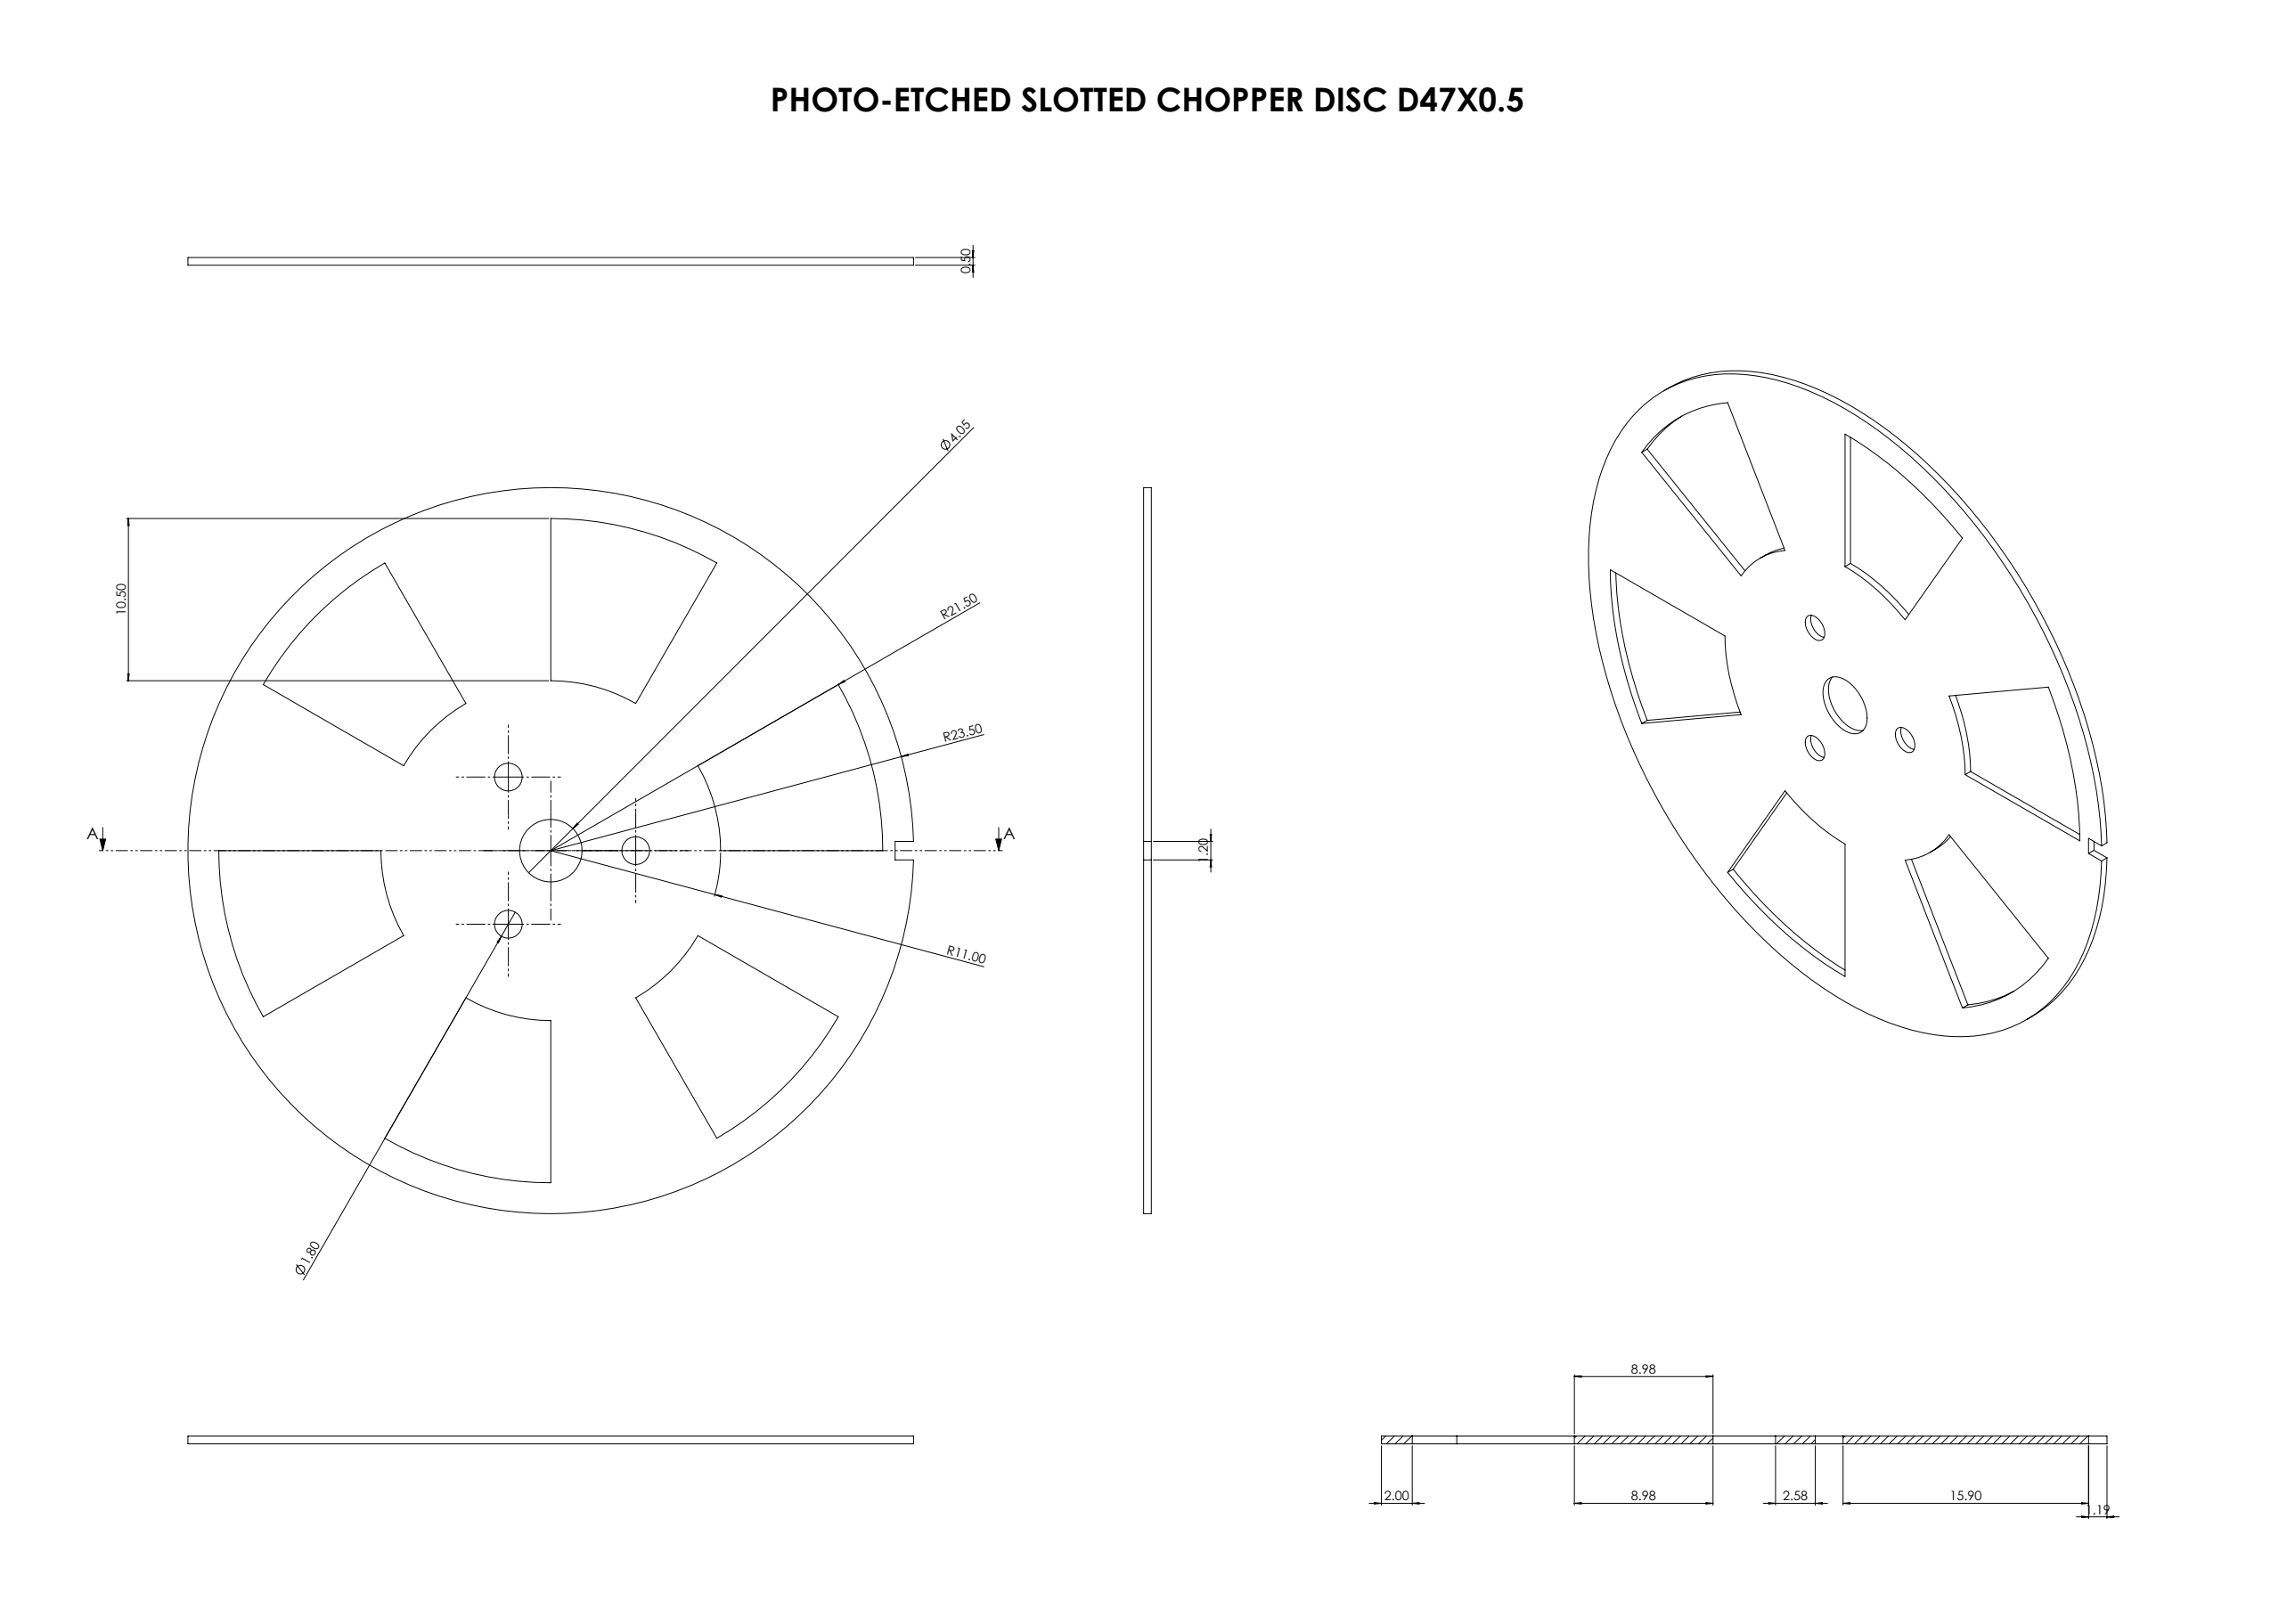
ISO-10303-21;
HEADER;
/* Generated by software containing ST-Developer
 * from STEP Tools, Inc. (www.steptools.com) 
 */

FILE_DESCRIPTION(
/* description */ (''),
/* implementation_level */ '2;1');

FILE_NAME(
/* name */ '10_Photo-Etched_Slotted_Chopper_Disc_D47x0.5.step',
/* time_stamp */ '2026-10-19T23:00:43-07:00',
/* author */ (''),
/* organization */ (''),
/* preprocessor_version */ 'ST-DEVELOPER v20.2',
/* originating_system */ 'Autodesk Translation Framework v15.15.0.0',
/* authorisation */ '');

FILE_SCHEMA (('AUTOMOTIVE_DESIGN { 1 0 10303 214 3 1 1 }'));
ENDSEC;

DATA;
#10=MECHANICAL_DESIGN_GEOMETRIC_PRESENTATION_REPRESENTATION('',(#1005),#55002);
#965=SHAPE_REPRESENTATION_RELATIONSHIP('SRR','None',#55113,#985);
#985=ADVANCED_BREP_SHAPE_REPRESENTATION('',(#1025),#54991);
#1005=STYLED_ITEM('',(#55379),#1025);
#1025=MANIFOLD_SOLID_BREP('Chopper Disc',#24538);
#1212=FACE_BOUND('',#4510,.T.);
#1213=FACE_BOUND('',#4511,.T.);
#1214=FACE_BOUND('',#4512,.T.);
#1215=FACE_BOUND('',#4513,.T.);
#1216=FACE_BOUND('',#4514,.T.);
#1217=FACE_BOUND('',#4515,.T.);
#1218=FACE_BOUND('',#4516,.T.);
#1219=FACE_BOUND('',#4517,.T.);
#1220=FACE_BOUND('',#4518,.T.);
#1221=FACE_BOUND('',#4519,.T.);
#1222=FACE_BOUND('',#4550,.T.);
#1223=FACE_BOUND('',#4551,.T.);
#1224=FACE_BOUND('',#4552,.T.);
#1225=FACE_BOUND('',#4553,.T.);
#1226=FACE_BOUND('',#4554,.T.);
#1227=FACE_BOUND('',#4555,.T.);
#1228=FACE_BOUND('',#4556,.T.);
#1229=FACE_BOUND('',#4557,.T.);
#1230=FACE_BOUND('',#4558,.T.);
#1231=FACE_BOUND('',#4559,.T.);
#1441=PLANE('',#25954);
#1442=PLANE('',#25955);
#1443=PLANE('',#25956);
#1444=PLANE('',#25957);
#1445=PLANE('',#25983);
#1446=PLANE('',#25986);
#1447=PLANE('',#25989);
#1448=PLANE('',#25992);
#1449=PLANE('',#25995);
#1450=PLANE('',#25998);
#1451=PLANE('',#26001);
#1452=PLANE('',#26004);
#1453=PLANE('',#26007);
#1454=PLANE('',#26010);
#1455=PLANE('',#26013);
#1456=PLANE('',#26016);
#1457=PLANE('',#26021);
#2161=CYLINDRICAL_SURFACE('',#25975,2.35);
#2162=CYLINDRICAL_SURFACE('',#25977,0.09);
#2163=CYLINDRICAL_SURFACE('',#25979,0.09);
#2164=CYLINDRICAL_SURFACE('',#25981,0.0900000000000001);
#2165=CYLINDRICAL_SURFACE('',#25984,1.1);
#2166=CYLINDRICAL_SURFACE('',#25987,2.15);
#2167=CYLINDRICAL_SURFACE('',#25990,1.1);
#2168=CYLINDRICAL_SURFACE('',#25993,2.15);
#2169=CYLINDRICAL_SURFACE('',#25996,1.1);
#2170=CYLINDRICAL_SURFACE('',#25999,2.15);
#2171=CYLINDRICAL_SURFACE('',#26002,1.1);
#2172=CYLINDRICAL_SURFACE('',#26005,2.15);
#2173=CYLINDRICAL_SURFACE('',#26008,1.1);
#2174=CYLINDRICAL_SURFACE('',#26011,2.15);
#2175=CYLINDRICAL_SURFACE('',#26014,1.1);
#2176=CYLINDRICAL_SURFACE('',#26017,2.15);
#2177=CYLINDRICAL_SURFACE('',#26019,0.2025);
#2966=FACE_OUTER_BOUND('',#4506,.T.);
#2967=FACE_OUTER_BOUND('',#4507,.T.);
#2968=FACE_OUTER_BOUND('',#4508,.T.);
#2969=FACE_OUTER_BOUND('',#4509,.T.);
#2970=FACE_OUTER_BOUND('',#4520,.T.);
#2971=FACE_OUTER_BOUND('',#4521,.T.);
#2972=FACE_OUTER_BOUND('',#4522,.T.);
#2973=FACE_OUTER_BOUND('',#4523,.T.);
#2974=FACE_OUTER_BOUND('',#4524,.T.);
#2975=FACE_OUTER_BOUND('',#4525,.T.);
#2976=FACE_OUTER_BOUND('',#4526,.T.);
#2977=FACE_OUTER_BOUND('',#4527,.T.);
#2978=FACE_OUTER_BOUND('',#4528,.T.);
#2979=FACE_OUTER_BOUND('',#4529,.T.);
#2980=FACE_OUTER_BOUND('',#4530,.T.);
#2981=FACE_OUTER_BOUND('',#4531,.T.);
#2982=FACE_OUTER_BOUND('',#4532,.T.);
#2983=FACE_OUTER_BOUND('',#4533,.T.);
#2984=FACE_OUTER_BOUND('',#4534,.T.);
#2985=FACE_OUTER_BOUND('',#4535,.T.);
#2986=FACE_OUTER_BOUND('',#4536,.T.);
#2987=FACE_OUTER_BOUND('',#4537,.T.);
#2988=FACE_OUTER_BOUND('',#4538,.T.);
#2989=FACE_OUTER_BOUND('',#4539,.T.);
#2990=FACE_OUTER_BOUND('',#4540,.T.);
#2991=FACE_OUTER_BOUND('',#4541,.T.);
#2992=FACE_OUTER_BOUND('',#4542,.T.);
#2993=FACE_OUTER_BOUND('',#4543,.T.);
#2994=FACE_OUTER_BOUND('',#4544,.T.);
#2995=FACE_OUTER_BOUND('',#4545,.T.);
#2996=FACE_OUTER_BOUND('',#4546,.T.);
#2997=FACE_OUTER_BOUND('',#4547,.T.);
#2998=FACE_OUTER_BOUND('',#4548,.T.);
#2999=FACE_OUTER_BOUND('',#4549,.T.);
#4506=EDGE_LOOP('',(#18412,#18413,#18414,#18415));
#4507=EDGE_LOOP('',(#18416,#18417,#18418,#18419));
#4508=EDGE_LOOP('',(#18420,#18421,#18422,#18423));
#4509=EDGE_LOOP('',(#18424,#18425,#18426,#18427));
#4510=EDGE_LOOP('',(#18428));
#4511=EDGE_LOOP('',(#18429));
#4512=EDGE_LOOP('',(#18430));
#4513=EDGE_LOOP('',(#18431,#18432,#18433,#18434));
#4514=EDGE_LOOP('',(#18435,#18436,#18437,#18438));
#4515=EDGE_LOOP('',(#18439,#18440,#18441,#18442));
#4516=EDGE_LOOP('',(#18443,#18444,#18445,#18446));
#4517=EDGE_LOOP('',(#18447,#18448,#18449,#18450));
#4518=EDGE_LOOP('',(#18451,#18452,#18453,#18454));
#4519=EDGE_LOOP('',(#18455));
#4520=EDGE_LOOP('',(#18456,#18457,#18458,#18459));
#4521=EDGE_LOOP('',(#18460,#18461,#18462,#18463));
#4522=EDGE_LOOP('',(#18464,#18465,#18466,#18467));
#4523=EDGE_LOOP('',(#18468,#18469,#18470,#18471));
#4524=EDGE_LOOP('',(#18472,#18473,#18474,#18475));
#4525=EDGE_LOOP('',(#18476,#18477,#18478,#18479));
#4526=EDGE_LOOP('',(#18480,#18481,#18482,#18483));
#4527=EDGE_LOOP('',(#18484,#18485,#18486,#18487));
#4528=EDGE_LOOP('',(#18488,#18489,#18490,#18491));
#4529=EDGE_LOOP('',(#18492,#18493,#18494,#18495));
#4530=EDGE_LOOP('',(#18496,#18497,#18498,#18499));
#4531=EDGE_LOOP('',(#18500,#18501,#18502,#18503));
#4532=EDGE_LOOP('',(#18504,#18505,#18506,#18507));
#4533=EDGE_LOOP('',(#18508,#18509,#18510,#18511));
#4534=EDGE_LOOP('',(#18512,#18513,#18514,#18515));
#4535=EDGE_LOOP('',(#18516,#18517,#18518,#18519));
#4536=EDGE_LOOP('',(#18520,#18521,#18522,#18523));
#4537=EDGE_LOOP('',(#18524,#18525,#18526,#18527));
#4538=EDGE_LOOP('',(#18528,#18529,#18530,#18531));
#4539=EDGE_LOOP('',(#18532,#18533,#18534,#18535));
#4540=EDGE_LOOP('',(#18536,#18537,#18538,#18539));
#4541=EDGE_LOOP('',(#18540,#18541,#18542,#18543));
#4542=EDGE_LOOP('',(#18544,#18545,#18546,#18547));
#4543=EDGE_LOOP('',(#18548,#18549,#18550,#18551));
#4544=EDGE_LOOP('',(#18552,#18553,#18554,#18555));
#4545=EDGE_LOOP('',(#18556,#18557,#18558,#18559));
#4546=EDGE_LOOP('',(#18560,#18561,#18562,#18563));
#4547=EDGE_LOOP('',(#18564,#18565,#18566,#18567));
#4548=EDGE_LOOP('',(#18568,#18569,#18570,#18571));
#4549=EDGE_LOOP('',(#18572,#18573,#18574,#18575));
#4550=EDGE_LOOP('',(#18576));
#4551=EDGE_LOOP('',(#18577));
#4552=EDGE_LOOP('',(#18578));
#4553=EDGE_LOOP('',(#18579,#18580,#18581,#18582));
#4554=EDGE_LOOP('',(#18583,#18584,#18585,#18586));
#4555=EDGE_LOOP('',(#18587,#18588,#18589,#18590));
#4556=EDGE_LOOP('',(#18591,#18592,#18593,#18594));
#4557=EDGE_LOOP('',(#18595,#18596,#18597,#18598));
#4558=EDGE_LOOP('',(#18599,#18600,#18601,#18602));
#4559=EDGE_LOOP('',(#18603));
#6000=LINE('',#37069,#7821);
#6001=LINE('',#37071,#7822);
#6002=LINE('',#37073,#7823);
#6003=LINE('',#37074,#7824);
#6004=LINE('',#37078,#7825);
#6005=LINE('',#37080,#7826);
#6006=LINE('',#37082,#7827);
#6007=LINE('',#37083,#7828);
#6008=LINE('',#37085,#7829);
#6009=LINE('',#37086,#7830);
#6010=LINE('',#37097,#7831);
#6011=LINE('',#37101,#7832);
#6012=LINE('',#37105,#7833);
#6013=LINE('',#37109,#7834);
#6014=LINE('',#37113,#7835);
#6015=LINE('',#37117,#7836);
#6016=LINE('',#37121,#7837);
#6017=LINE('',#37125,#7838);
#6018=LINE('',#37129,#7839);
#6019=LINE('',#37133,#7840);
#6020=LINE('',#37137,#7841);
#6021=LINE('',#37141,#7842);
#6022=LINE('',#37150,#7843);
#6023=LINE('',#37154,#7844);
#6024=LINE('',#37158,#7845);
#6025=LINE('',#37161,#7846);
#6026=LINE('',#37163,#7847);
#6027=LINE('',#37164,#7848);
#6028=LINE('',#37167,#7849);
#6029=LINE('',#37171,#7850);
#6030=LINE('',#37172,#7851);
#6031=LINE('',#37177,#7852);
#6032=LINE('',#37179,#7853);
#6033=LINE('',#37180,#7854);
#6034=LINE('',#37183,#7855);
#6035=LINE('',#37187,#7856);
#6036=LINE('',#37188,#7857);
#6037=LINE('',#37193,#7858);
#6038=LINE('',#37195,#7859);
#6039=LINE('',#37196,#7860);
#6040=LINE('',#37199,#7861);
#6041=LINE('',#37203,#7862);
#6042=LINE('',#37204,#7863);
#6043=LINE('',#37209,#7864);
#6044=LINE('',#37211,#7865);
#6045=LINE('',#37212,#7866);
#6046=LINE('',#37215,#7867);
#6047=LINE('',#37219,#7868);
#6048=LINE('',#37220,#7869);
#6049=LINE('',#37225,#7870);
#6050=LINE('',#37227,#7871);
#6051=LINE('',#37228,#7872);
#6052=LINE('',#37231,#7873);
#6053=LINE('',#37235,#7874);
#6054=LINE('',#37236,#7875);
#6055=LINE('',#37241,#7876);
#6056=LINE('',#37243,#7877);
#6057=LINE('',#37244,#7878);
#6058=LINE('',#37247,#7879);
#6059=LINE('',#37251,#7880);
#6060=LINE('',#37252,#7881);
#6061=LINE('',#37258,#7882);
#7821=VECTOR('',#30186,1.);
#7822=VECTOR('',#30187,1.);
#7823=VECTOR('',#30188,1.);
#7824=VECTOR('',#30189,1.);
#7825=VECTOR('',#30192,1.);
#7826=VECTOR('',#30193,1.);
#7827=VECTOR('',#30194,1.);
#7828=VECTOR('',#30195,1.);
#7829=VECTOR('',#30198,1.);
#7830=VECTOR('',#30199,1.);
#7831=VECTOR('',#30210,1.);
#7832=VECTOR('',#30213,1.);
#7833=VECTOR('',#30216,1.);
#7834=VECTOR('',#30219,1.);
#7835=VECTOR('',#30222,1.);
#7836=VECTOR('',#30225,1.);
#7837=VECTOR('',#30228,1.);
#7838=VECTOR('',#30231,1.);
#7839=VECTOR('',#30234,1.);
#7840=VECTOR('',#30237,1.);
#7841=VECTOR('',#30240,1.);
#7842=VECTOR('',#30243,1.);
#7843=VECTOR('',#30256,0.09);
#7844=VECTOR('',#30261,0.09);
#7845=VECTOR('',#30266,0.0900000000000001);
#7846=VECTOR('',#30269,1.);
#7847=VECTOR('',#30270,1.);
#7848=VECTOR('',#30271,1.);
#7849=VECTOR('',#30274,1.);
#7850=VECTOR('',#30279,1.);
#7851=VECTOR('',#30280,1.);
#7852=VECTOR('',#30287,1.);
#7853=VECTOR('',#30288,1.);
#7854=VECTOR('',#30289,1.);
#7855=VECTOR('',#30292,1.);
#7856=VECTOR('',#30297,1.);
#7857=VECTOR('',#30298,1.);
#7858=VECTOR('',#30305,1.);
#7859=VECTOR('',#30306,1.);
#7860=VECTOR('',#30307,1.);
#7861=VECTOR('',#30310,1.);
#7862=VECTOR('',#30315,1.);
#7863=VECTOR('',#30316,1.);
#7864=VECTOR('',#30323,1.);
#7865=VECTOR('',#30324,1.);
#7866=VECTOR('',#30325,1.);
#7867=VECTOR('',#30328,1.);
#7868=VECTOR('',#30333,1.);
#7869=VECTOR('',#30334,1.);
#7870=VECTOR('',#30341,1.);
#7871=VECTOR('',#30342,1.);
#7872=VECTOR('',#30343,1.);
#7873=VECTOR('',#30346,1.);
#7874=VECTOR('',#30351,1.);
#7875=VECTOR('',#30352,1.);
#7876=VECTOR('',#30359,1.);
#7877=VECTOR('',#30360,1.);
#7878=VECTOR('',#30361,1.);
#7879=VECTOR('',#30364,1.);
#7880=VECTOR('',#30369,1.);
#7881=VECTOR('',#30370,1.);
#7882=VECTOR('',#30379,0.2025);
#9644=CIRCLE('',#25958,2.35);
#9645=CIRCLE('',#25959,0.09);
#9646=CIRCLE('',#25960,0.0900000000000001);
#9647=CIRCLE('',#25961,0.2025);
#9648=CIRCLE('',#25962,2.15);
#9649=CIRCLE('',#25963,1.1);
#9650=CIRCLE('',#25964,2.15);
#9651=CIRCLE('',#25965,1.1);
#9652=CIRCLE('',#25966,2.15);
#9653=CIRCLE('',#25967,1.1);
#9654=CIRCLE('',#25968,2.15);
#9655=CIRCLE('',#25969,1.1);
#9656=CIRCLE('',#25970,2.15);
#9657=CIRCLE('',#25971,1.1);
#9658=CIRCLE('',#25972,2.15);
#9659=CIRCLE('',#25973,1.1);
#9660=CIRCLE('',#25974,0.09);
#9661=CIRCLE('',#25976,2.35);
#9662=CIRCLE('',#25978,0.09);
#9663=CIRCLE('',#25980,0.09);
#9664=CIRCLE('',#25982,0.0900000000000001);
#9665=CIRCLE('',#25985,1.1);
#9666=CIRCLE('',#25988,2.15);
#9667=CIRCLE('',#25991,1.1);
#9668=CIRCLE('',#25994,2.15);
#9669=CIRCLE('',#25997,1.1);
#9670=CIRCLE('',#26000,2.15);
#9671=CIRCLE('',#26003,1.1);
#9672=CIRCLE('',#26006,2.15);
#9673=CIRCLE('',#26009,1.1);
#9674=CIRCLE('',#26012,2.15);
#9675=CIRCLE('',#26015,1.1);
#9676=CIRCLE('',#26018,2.15);
#9677=CIRCLE('',#26020,0.2025);
#10841=VERTEX_POINT('',#37067);
#10842=VERTEX_POINT('',#37068);
#10843=VERTEX_POINT('',#37070);
#10844=VERTEX_POINT('',#37072);
#10845=VERTEX_POINT('',#37076);
#10846=VERTEX_POINT('',#37077);
#10847=VERTEX_POINT('',#37079);
#10848=VERTEX_POINT('',#37081);
#10849=VERTEX_POINT('',#37089);
#10850=VERTEX_POINT('',#37091);
#10851=VERTEX_POINT('',#37093);
#10852=VERTEX_POINT('',#37095);
#10853=VERTEX_POINT('',#37096);
#10854=VERTEX_POINT('',#37098);
#10855=VERTEX_POINT('',#37100);
#10856=VERTEX_POINT('',#37103);
#10857=VERTEX_POINT('',#37104);
#10858=VERTEX_POINT('',#37106);
#10859=VERTEX_POINT('',#37108);
#10860=VERTEX_POINT('',#37111);
#10861=VERTEX_POINT('',#37112);
#10862=VERTEX_POINT('',#37114);
#10863=VERTEX_POINT('',#37116);
#10864=VERTEX_POINT('',#37119);
#10865=VERTEX_POINT('',#37120);
#10866=VERTEX_POINT('',#37122);
#10867=VERTEX_POINT('',#37124);
#10868=VERTEX_POINT('',#37127);
#10869=VERTEX_POINT('',#37128);
#10870=VERTEX_POINT('',#37130);
#10871=VERTEX_POINT('',#37132);
#10872=VERTEX_POINT('',#37135);
#10873=VERTEX_POINT('',#37136);
#10874=VERTEX_POINT('',#37138);
#10875=VERTEX_POINT('',#37140);
#10876=VERTEX_POINT('',#37143);
#10877=VERTEX_POINT('',#37148);
#10878=VERTEX_POINT('',#37152);
#10879=VERTEX_POINT('',#37156);
#10880=VERTEX_POINT('',#37160);
#10881=VERTEX_POINT('',#37162);
#10882=VERTEX_POINT('',#37166);
#10883=VERTEX_POINT('',#37170);
#10884=VERTEX_POINT('',#37176);
#10885=VERTEX_POINT('',#37178);
#10886=VERTEX_POINT('',#37182);
#10887=VERTEX_POINT('',#37186);
#10888=VERTEX_POINT('',#37192);
#10889=VERTEX_POINT('',#37194);
#10890=VERTEX_POINT('',#37198);
#10891=VERTEX_POINT('',#37202);
#10892=VERTEX_POINT('',#37208);
#10893=VERTEX_POINT('',#37210);
#10894=VERTEX_POINT('',#37214);
#10895=VERTEX_POINT('',#37218);
#10896=VERTEX_POINT('',#37224);
#10897=VERTEX_POINT('',#37226);
#10898=VERTEX_POINT('',#37230);
#10899=VERTEX_POINT('',#37234);
#10900=VERTEX_POINT('',#37240);
#10901=VERTEX_POINT('',#37242);
#10902=VERTEX_POINT('',#37246);
#10903=VERTEX_POINT('',#37250);
#10904=VERTEX_POINT('',#37256);
#13614=EDGE_CURVE('',#10841,#10842,#6000,.T.);
#13615=EDGE_CURVE('',#10843,#10841,#6001,.T.);
#13616=EDGE_CURVE('',#10844,#10843,#6002,.T.);
#13617=EDGE_CURVE('',#10842,#10844,#6003,.T.);
#13618=EDGE_CURVE('',#10845,#10846,#6004,.T.);
#13619=EDGE_CURVE('',#10847,#10845,#6005,.T.);
#13620=EDGE_CURVE('',#10847,#10848,#6006,.T.);
#13621=EDGE_CURVE('',#10846,#10848,#6007,.T.);
#13622=EDGE_CURVE('',#10844,#10847,#6008,.T.);
#13623=EDGE_CURVE('',#10848,#10843,#6009,.T.);
#13624=EDGE_CURVE('',#10842,#10845,#9644,.T.);
#13625=EDGE_CURVE('',#10849,#10849,#9645,.T.);
#13626=EDGE_CURVE('',#10850,#10850,#9646,.T.);
#13627=EDGE_CURVE('',#10851,#10851,#9647,.T.);
#13628=EDGE_CURVE('',#10852,#10853,#6010,.T.);
#13629=EDGE_CURVE('',#10853,#10854,#9648,.T.);
#13630=EDGE_CURVE('',#10854,#10855,#6011,.T.);
#13631=EDGE_CURVE('',#10855,#10852,#9649,.T.);
#13632=EDGE_CURVE('',#10856,#10857,#6012,.T.);
#13633=EDGE_CURVE('',#10857,#10858,#9650,.T.);
#13634=EDGE_CURVE('',#10858,#10859,#6013,.T.);
#13635=EDGE_CURVE('',#10859,#10856,#9651,.T.);
#13636=EDGE_CURVE('',#10860,#10861,#6014,.T.);
#13637=EDGE_CURVE('',#10861,#10862,#9652,.T.);
#13638=EDGE_CURVE('',#10862,#10863,#6015,.T.);
#13639=EDGE_CURVE('',#10863,#10860,#9653,.T.);
#13640=EDGE_CURVE('',#10864,#10865,#6016,.T.);
#13641=EDGE_CURVE('',#10865,#10866,#9654,.T.);
#13642=EDGE_CURVE('',#10866,#10867,#6017,.T.);
#13643=EDGE_CURVE('',#10867,#10864,#9655,.T.);
#13644=EDGE_CURVE('',#10868,#10869,#6018,.T.);
#13645=EDGE_CURVE('',#10869,#10870,#9656,.T.);
#13646=EDGE_CURVE('',#10870,#10871,#6019,.T.);
#13647=EDGE_CURVE('',#10871,#10868,#9657,.T.);
#13648=EDGE_CURVE('',#10872,#10873,#6020,.T.);
#13649=EDGE_CURVE('',#10873,#10874,#9658,.T.);
#13650=EDGE_CURVE('',#10874,#10875,#6021,.T.);
#13651=EDGE_CURVE('',#10875,#10872,#9659,.T.);
#13652=EDGE_CURVE('',#10876,#10876,#9660,.T.);
#13653=EDGE_CURVE('',#10841,#10846,#9661,.T.);
#13654=EDGE_CURVE('',#10877,#10877,#9662,.T.);
#13655=EDGE_CURVE('',#10877,#10849,#6022,.T.);
#13656=EDGE_CURVE('',#10878,#10878,#9663,.T.);
#13657=EDGE_CURVE('',#10878,#10876,#6023,.T.);
#13658=EDGE_CURVE('',#10879,#10879,#9664,.T.);
#13659=EDGE_CURVE('',#10879,#10850,#6024,.T.);
#13660=EDGE_CURVE('',#10872,#10880,#6025,.T.);
#13661=EDGE_CURVE('',#10881,#10880,#6026,.T.);
#13662=EDGE_CURVE('',#10873,#10881,#6027,.T.);
#13663=EDGE_CURVE('',#10875,#10882,#6028,.T.);
#13664=EDGE_CURVE('',#10880,#10882,#9665,.T.);
#13665=EDGE_CURVE('',#10874,#10883,#6029,.T.);
#13666=EDGE_CURVE('',#10882,#10883,#6030,.T.);
#13667=EDGE_CURVE('',#10883,#10881,#9666,.T.);
#13668=EDGE_CURVE('',#10868,#10884,#6031,.T.);
#13669=EDGE_CURVE('',#10885,#10884,#6032,.T.);
#13670=EDGE_CURVE('',#10869,#10885,#6033,.T.);
#13671=EDGE_CURVE('',#10871,#10886,#6034,.T.);
#13672=EDGE_CURVE('',#10884,#10886,#9667,.T.);
#13673=EDGE_CURVE('',#10870,#10887,#6035,.T.);
#13674=EDGE_CURVE('',#10886,#10887,#6036,.T.);
#13675=EDGE_CURVE('',#10887,#10885,#9668,.T.);
#13676=EDGE_CURVE('',#10864,#10888,#6037,.T.);
#13677=EDGE_CURVE('',#10889,#10888,#6038,.T.);
#13678=EDGE_CURVE('',#10865,#10889,#6039,.T.);
#13679=EDGE_CURVE('',#10867,#10890,#6040,.T.);
#13680=EDGE_CURVE('',#10888,#10890,#9669,.T.);
#13681=EDGE_CURVE('',#10866,#10891,#6041,.T.);
#13682=EDGE_CURVE('',#10890,#10891,#6042,.T.);
#13683=EDGE_CURVE('',#10891,#10889,#9670,.T.);
#13684=EDGE_CURVE('',#10860,#10892,#6043,.T.);
#13685=EDGE_CURVE('',#10893,#10892,#6044,.T.);
#13686=EDGE_CURVE('',#10861,#10893,#6045,.T.);
#13687=EDGE_CURVE('',#10863,#10894,#6046,.T.);
#13688=EDGE_CURVE('',#10892,#10894,#9671,.T.);
#13689=EDGE_CURVE('',#10862,#10895,#6047,.T.);
#13690=EDGE_CURVE('',#10894,#10895,#6048,.T.);
#13691=EDGE_CURVE('',#10895,#10893,#9672,.T.);
#13692=EDGE_CURVE('',#10856,#10896,#6049,.T.);
#13693=EDGE_CURVE('',#10897,#10896,#6050,.T.);
#13694=EDGE_CURVE('',#10857,#10897,#6051,.T.);
#13695=EDGE_CURVE('',#10859,#10898,#6052,.T.);
#13696=EDGE_CURVE('',#10896,#10898,#9673,.T.);
#13697=EDGE_CURVE('',#10858,#10899,#6053,.T.);
#13698=EDGE_CURVE('',#10898,#10899,#6054,.T.);
#13699=EDGE_CURVE('',#10899,#10897,#9674,.T.);
#13700=EDGE_CURVE('',#10852,#10900,#6055,.T.);
#13701=EDGE_CURVE('',#10901,#10900,#6056,.T.);
#13702=EDGE_CURVE('',#10853,#10901,#6057,.T.);
#13703=EDGE_CURVE('',#10855,#10902,#6058,.T.);
#13704=EDGE_CURVE('',#10900,#10902,#9675,.T.);
#13705=EDGE_CURVE('',#10854,#10903,#6059,.T.);
#13706=EDGE_CURVE('',#10902,#10903,#6060,.T.);
#13707=EDGE_CURVE('',#10903,#10901,#9676,.T.);
#13708=EDGE_CURVE('',#10904,#10904,#9677,.T.);
#13709=EDGE_CURVE('',#10904,#10851,#6061,.T.);
#18412=ORIENTED_EDGE('',*,*,#13614,.F.);
#18413=ORIENTED_EDGE('',*,*,#13615,.F.);
#18414=ORIENTED_EDGE('',*,*,#13616,.F.);
#18415=ORIENTED_EDGE('',*,*,#13617,.F.);
#18416=ORIENTED_EDGE('',*,*,#13618,.F.);
#18417=ORIENTED_EDGE('',*,*,#13619,.F.);
#18418=ORIENTED_EDGE('',*,*,#13620,.T.);
#18419=ORIENTED_EDGE('',*,*,#13621,.F.);
#18420=ORIENTED_EDGE('',*,*,#13622,.F.);
#18421=ORIENTED_EDGE('',*,*,#13616,.T.);
#18422=ORIENTED_EDGE('',*,*,#13623,.F.);
#18423=ORIENTED_EDGE('',*,*,#13620,.F.);
#18424=ORIENTED_EDGE('',*,*,#13617,.T.);
#18425=ORIENTED_EDGE('',*,*,#13622,.T.);
#18426=ORIENTED_EDGE('',*,*,#13619,.T.);
#18427=ORIENTED_EDGE('',*,*,#13624,.F.);
#18428=ORIENTED_EDGE('',*,*,#13625,.T.);
#18429=ORIENTED_EDGE('',*,*,#13626,.T.);
#18430=ORIENTED_EDGE('',*,*,#13627,.T.);
#18431=ORIENTED_EDGE('',*,*,#13628,.T.);
#18432=ORIENTED_EDGE('',*,*,#13629,.T.);
#18433=ORIENTED_EDGE('',*,*,#13630,.T.);
#18434=ORIENTED_EDGE('',*,*,#13631,.T.);
#18435=ORIENTED_EDGE('',*,*,#13632,.T.);
#18436=ORIENTED_EDGE('',*,*,#13633,.T.);
#18437=ORIENTED_EDGE('',*,*,#13634,.T.);
#18438=ORIENTED_EDGE('',*,*,#13635,.T.);
#18439=ORIENTED_EDGE('',*,*,#13636,.T.);
#18440=ORIENTED_EDGE('',*,*,#13637,.T.);
#18441=ORIENTED_EDGE('',*,*,#13638,.T.);
#18442=ORIENTED_EDGE('',*,*,#13639,.T.);
#18443=ORIENTED_EDGE('',*,*,#13640,.T.);
#18444=ORIENTED_EDGE('',*,*,#13641,.T.);
#18445=ORIENTED_EDGE('',*,*,#13642,.T.);
#18446=ORIENTED_EDGE('',*,*,#13643,.T.);
#18447=ORIENTED_EDGE('',*,*,#13644,.T.);
#18448=ORIENTED_EDGE('',*,*,#13645,.T.);
#18449=ORIENTED_EDGE('',*,*,#13646,.T.);
#18450=ORIENTED_EDGE('',*,*,#13647,.T.);
#18451=ORIENTED_EDGE('',*,*,#13648,.T.);
#18452=ORIENTED_EDGE('',*,*,#13649,.T.);
#18453=ORIENTED_EDGE('',*,*,#13650,.T.);
#18454=ORIENTED_EDGE('',*,*,#13651,.T.);
#18455=ORIENTED_EDGE('',*,*,#13652,.T.);
#18456=ORIENTED_EDGE('',*,*,#13614,.T.);
#18457=ORIENTED_EDGE('',*,*,#13624,.T.);
#18458=ORIENTED_EDGE('',*,*,#13618,.T.);
#18459=ORIENTED_EDGE('',*,*,#13653,.F.);
#18460=ORIENTED_EDGE('',*,*,#13654,.F.);
#18461=ORIENTED_EDGE('',*,*,#13655,.T.);
#18462=ORIENTED_EDGE('',*,*,#13625,.F.);
#18463=ORIENTED_EDGE('',*,*,#13655,.F.);
#18464=ORIENTED_EDGE('',*,*,#13656,.F.);
#18465=ORIENTED_EDGE('',*,*,#13657,.T.);
#18466=ORIENTED_EDGE('',*,*,#13652,.F.);
#18467=ORIENTED_EDGE('',*,*,#13657,.F.);
#18468=ORIENTED_EDGE('',*,*,#13658,.F.);
#18469=ORIENTED_EDGE('',*,*,#13659,.T.);
#18470=ORIENTED_EDGE('',*,*,#13626,.F.);
#18471=ORIENTED_EDGE('',*,*,#13659,.F.);
#18472=ORIENTED_EDGE('',*,*,#13648,.F.);
#18473=ORIENTED_EDGE('',*,*,#13660,.T.);
#18474=ORIENTED_EDGE('',*,*,#13661,.F.);
#18475=ORIENTED_EDGE('',*,*,#13662,.F.);
#18476=ORIENTED_EDGE('',*,*,#13651,.F.);
#18477=ORIENTED_EDGE('',*,*,#13663,.T.);
#18478=ORIENTED_EDGE('',*,*,#13664,.F.);
#18479=ORIENTED_EDGE('',*,*,#13660,.F.);
#18480=ORIENTED_EDGE('',*,*,#13650,.F.);
#18481=ORIENTED_EDGE('',*,*,#13665,.T.);
#18482=ORIENTED_EDGE('',*,*,#13666,.F.);
#18483=ORIENTED_EDGE('',*,*,#13663,.F.);
#18484=ORIENTED_EDGE('',*,*,#13649,.F.);
#18485=ORIENTED_EDGE('',*,*,#13662,.T.);
#18486=ORIENTED_EDGE('',*,*,#13667,.F.);
#18487=ORIENTED_EDGE('',*,*,#13665,.F.);
#18488=ORIENTED_EDGE('',*,*,#13644,.F.);
#18489=ORIENTED_EDGE('',*,*,#13668,.T.);
#18490=ORIENTED_EDGE('',*,*,#13669,.F.);
#18491=ORIENTED_EDGE('',*,*,#13670,.F.);
#18492=ORIENTED_EDGE('',*,*,#13647,.F.);
#18493=ORIENTED_EDGE('',*,*,#13671,.T.);
#18494=ORIENTED_EDGE('',*,*,#13672,.F.);
#18495=ORIENTED_EDGE('',*,*,#13668,.F.);
#18496=ORIENTED_EDGE('',*,*,#13646,.F.);
#18497=ORIENTED_EDGE('',*,*,#13673,.T.);
#18498=ORIENTED_EDGE('',*,*,#13674,.F.);
#18499=ORIENTED_EDGE('',*,*,#13671,.F.);
#18500=ORIENTED_EDGE('',*,*,#13645,.F.);
#18501=ORIENTED_EDGE('',*,*,#13670,.T.);
#18502=ORIENTED_EDGE('',*,*,#13675,.F.);
#18503=ORIENTED_EDGE('',*,*,#13673,.F.);
#18504=ORIENTED_EDGE('',*,*,#13640,.F.);
#18505=ORIENTED_EDGE('',*,*,#13676,.T.);
#18506=ORIENTED_EDGE('',*,*,#13677,.F.);
#18507=ORIENTED_EDGE('',*,*,#13678,.F.);
#18508=ORIENTED_EDGE('',*,*,#13643,.F.);
#18509=ORIENTED_EDGE('',*,*,#13679,.T.);
#18510=ORIENTED_EDGE('',*,*,#13680,.F.);
#18511=ORIENTED_EDGE('',*,*,#13676,.F.);
#18512=ORIENTED_EDGE('',*,*,#13642,.F.);
#18513=ORIENTED_EDGE('',*,*,#13681,.T.);
#18514=ORIENTED_EDGE('',*,*,#13682,.F.);
#18515=ORIENTED_EDGE('',*,*,#13679,.F.);
#18516=ORIENTED_EDGE('',*,*,#13641,.F.);
#18517=ORIENTED_EDGE('',*,*,#13678,.T.);
#18518=ORIENTED_EDGE('',*,*,#13683,.F.);
#18519=ORIENTED_EDGE('',*,*,#13681,.F.);
#18520=ORIENTED_EDGE('',*,*,#13636,.F.);
#18521=ORIENTED_EDGE('',*,*,#13684,.T.);
#18522=ORIENTED_EDGE('',*,*,#13685,.F.);
#18523=ORIENTED_EDGE('',*,*,#13686,.F.);
#18524=ORIENTED_EDGE('',*,*,#13639,.F.);
#18525=ORIENTED_EDGE('',*,*,#13687,.T.);
#18526=ORIENTED_EDGE('',*,*,#13688,.F.);
#18527=ORIENTED_EDGE('',*,*,#13684,.F.);
#18528=ORIENTED_EDGE('',*,*,#13638,.F.);
#18529=ORIENTED_EDGE('',*,*,#13689,.T.);
#18530=ORIENTED_EDGE('',*,*,#13690,.F.);
#18531=ORIENTED_EDGE('',*,*,#13687,.F.);
#18532=ORIENTED_EDGE('',*,*,#13637,.F.);
#18533=ORIENTED_EDGE('',*,*,#13686,.T.);
#18534=ORIENTED_EDGE('',*,*,#13691,.F.);
#18535=ORIENTED_EDGE('',*,*,#13689,.F.);
#18536=ORIENTED_EDGE('',*,*,#13632,.F.);
#18537=ORIENTED_EDGE('',*,*,#13692,.T.);
#18538=ORIENTED_EDGE('',*,*,#13693,.F.);
#18539=ORIENTED_EDGE('',*,*,#13694,.F.);
#18540=ORIENTED_EDGE('',*,*,#13635,.F.);
#18541=ORIENTED_EDGE('',*,*,#13695,.T.);
#18542=ORIENTED_EDGE('',*,*,#13696,.F.);
#18543=ORIENTED_EDGE('',*,*,#13692,.F.);
#18544=ORIENTED_EDGE('',*,*,#13634,.F.);
#18545=ORIENTED_EDGE('',*,*,#13697,.T.);
#18546=ORIENTED_EDGE('',*,*,#13698,.F.);
#18547=ORIENTED_EDGE('',*,*,#13695,.F.);
#18548=ORIENTED_EDGE('',*,*,#13633,.F.);
#18549=ORIENTED_EDGE('',*,*,#13694,.T.);
#18550=ORIENTED_EDGE('',*,*,#13699,.F.);
#18551=ORIENTED_EDGE('',*,*,#13697,.F.);
#18552=ORIENTED_EDGE('',*,*,#13628,.F.);
#18553=ORIENTED_EDGE('',*,*,#13700,.T.);
#18554=ORIENTED_EDGE('',*,*,#13701,.F.);
#18555=ORIENTED_EDGE('',*,*,#13702,.F.);
#18556=ORIENTED_EDGE('',*,*,#13631,.F.);
#18557=ORIENTED_EDGE('',*,*,#13703,.T.);
#18558=ORIENTED_EDGE('',*,*,#13704,.F.);
#18559=ORIENTED_EDGE('',*,*,#13700,.F.);
#18560=ORIENTED_EDGE('',*,*,#13630,.F.);
#18561=ORIENTED_EDGE('',*,*,#13705,.T.);
#18562=ORIENTED_EDGE('',*,*,#13706,.F.);
#18563=ORIENTED_EDGE('',*,*,#13703,.F.);
#18564=ORIENTED_EDGE('',*,*,#13629,.F.);
#18565=ORIENTED_EDGE('',*,*,#13702,.T.);
#18566=ORIENTED_EDGE('',*,*,#13707,.F.);
#18567=ORIENTED_EDGE('',*,*,#13705,.F.);
#18568=ORIENTED_EDGE('',*,*,#13708,.T.);
#18569=ORIENTED_EDGE('',*,*,#13709,.T.);
#18570=ORIENTED_EDGE('',*,*,#13627,.F.);
#18571=ORIENTED_EDGE('',*,*,#13709,.F.);
#18572=ORIENTED_EDGE('',*,*,#13615,.T.);
#18573=ORIENTED_EDGE('',*,*,#13653,.T.);
#18574=ORIENTED_EDGE('',*,*,#13621,.T.);
#18575=ORIENTED_EDGE('',*,*,#13623,.T.);
#18576=ORIENTED_EDGE('',*,*,#13654,.T.);
#18577=ORIENTED_EDGE('',*,*,#13658,.T.);
#18578=ORIENTED_EDGE('',*,*,#13708,.F.);
#18579=ORIENTED_EDGE('',*,*,#13701,.T.);
#18580=ORIENTED_EDGE('',*,*,#13704,.T.);
#18581=ORIENTED_EDGE('',*,*,#13706,.T.);
#18582=ORIENTED_EDGE('',*,*,#13707,.T.);
#18583=ORIENTED_EDGE('',*,*,#13693,.T.);
#18584=ORIENTED_EDGE('',*,*,#13696,.T.);
#18585=ORIENTED_EDGE('',*,*,#13698,.T.);
#18586=ORIENTED_EDGE('',*,*,#13699,.T.);
#18587=ORIENTED_EDGE('',*,*,#13685,.T.);
#18588=ORIENTED_EDGE('',*,*,#13688,.T.);
#18589=ORIENTED_EDGE('',*,*,#13690,.T.);
#18590=ORIENTED_EDGE('',*,*,#13691,.T.);
#18591=ORIENTED_EDGE('',*,*,#13677,.T.);
#18592=ORIENTED_EDGE('',*,*,#13680,.T.);
#18593=ORIENTED_EDGE('',*,*,#13682,.T.);
#18594=ORIENTED_EDGE('',*,*,#13683,.T.);
#18595=ORIENTED_EDGE('',*,*,#13669,.T.);
#18596=ORIENTED_EDGE('',*,*,#13672,.T.);
#18597=ORIENTED_EDGE('',*,*,#13674,.T.);
#18598=ORIENTED_EDGE('',*,*,#13675,.T.);
#18599=ORIENTED_EDGE('',*,*,#13661,.T.);
#18600=ORIENTED_EDGE('',*,*,#13664,.T.);
#18601=ORIENTED_EDGE('',*,*,#13666,.T.);
#18602=ORIENTED_EDGE('',*,*,#13667,.T.);
#18603=ORIENTED_EDGE('',*,*,#13656,.T.);
#23719=ADVANCED_FACE('',(#2966),#1441,.F.);
#23720=ADVANCED_FACE('',(#2967),#1442,.F.);
#23721=ADVANCED_FACE('',(#2968),#1443,.F.);
#23722=ADVANCED_FACE('',(#2969,#1212,#1213,#1214,#1215,#1216,#1217,#1218,
#1219,#1220,#1221),#1444,.T.);
#23723=ADVANCED_FACE('',(#2970),#2161,.T.);
#23724=ADVANCED_FACE('',(#2971),#2162,.F.);
#23725=ADVANCED_FACE('',(#2972),#2163,.F.);
#23726=ADVANCED_FACE('',(#2973),#2164,.F.);
#23727=ADVANCED_FACE('',(#2974),#1445,.F.);
#23728=ADVANCED_FACE('',(#2975),#2165,.T.);
#23729=ADVANCED_FACE('',(#2976),#1446,.F.);
#23730=ADVANCED_FACE('',(#2977),#2166,.F.);
#23731=ADVANCED_FACE('',(#2978),#1447,.F.);
#23732=ADVANCED_FACE('',(#2979),#2167,.T.);
#23733=ADVANCED_FACE('',(#2980),#1448,.F.);
#23734=ADVANCED_FACE('',(#2981),#2168,.F.);
#23735=ADVANCED_FACE('',(#2982),#1449,.F.);
#23736=ADVANCED_FACE('',(#2983),#2169,.T.);
#23737=ADVANCED_FACE('',(#2984),#1450,.F.);
#23738=ADVANCED_FACE('',(#2985),#2170,.F.);
#23739=ADVANCED_FACE('',(#2986),#1451,.F.);
#23740=ADVANCED_FACE('',(#2987),#2171,.T.);
#23741=ADVANCED_FACE('',(#2988),#1452,.F.);
#23742=ADVANCED_FACE('',(#2989),#2172,.F.);
#23743=ADVANCED_FACE('',(#2990),#1453,.F.);
#23744=ADVANCED_FACE('',(#2991),#2173,.T.);
#23745=ADVANCED_FACE('',(#2992),#1454,.F.);
#23746=ADVANCED_FACE('',(#2993),#2174,.F.);
#23747=ADVANCED_FACE('',(#2994),#1455,.F.);
#23748=ADVANCED_FACE('',(#2995),#2175,.T.);
#23749=ADVANCED_FACE('',(#2996),#1456,.F.);
#23750=ADVANCED_FACE('',(#2997),#2176,.F.);
#23751=ADVANCED_FACE('',(#2998),#2177,.F.);
#23752=ADVANCED_FACE('',(#2999,#1222,#1223,#1224,#1225,#1226,#1227,#1228,
#1229,#1230,#1231),#1457,.T.);
#24538=CLOSED_SHELL('',(#23719,#23720,#23721,#23722,#23723,#23724,#23725,
#23726,#23727,#23728,#23729,#23730,#23731,#23732,#23733,#23734,#23735,#23736,
#23737,#23738,#23739,#23740,#23741,#23742,#23743,#23744,#23745,#23746,#23747,
#23748,#23749,#23750,#23751,#23752));
#25953=AXIS2_PLACEMENT_3D('',#37065,#30182,#30183);
#25954=AXIS2_PLACEMENT_3D('',#37066,#30184,#30185);
#25955=AXIS2_PLACEMENT_3D('',#37075,#30190,#30191);
#25956=AXIS2_PLACEMENT_3D('',#37084,#30196,#30197);
#25957=AXIS2_PLACEMENT_3D('',#37087,#30200,#30201);
#25958=AXIS2_PLACEMENT_3D('',#37088,#30202,#30203);
#25959=AXIS2_PLACEMENT_3D('',#37090,#30204,#30205);
#25960=AXIS2_PLACEMENT_3D('',#37092,#30206,#30207);
#25961=AXIS2_PLACEMENT_3D('',#37094,#30208,#30209);
#25962=AXIS2_PLACEMENT_3D('',#37099,#30211,#30212);
#25963=AXIS2_PLACEMENT_3D('',#37102,#30214,#30215);
#25964=AXIS2_PLACEMENT_3D('',#37107,#30217,#30218);
#25965=AXIS2_PLACEMENT_3D('',#37110,#30220,#30221);
#25966=AXIS2_PLACEMENT_3D('',#37115,#30223,#30224);
#25967=AXIS2_PLACEMENT_3D('',#37118,#30226,#30227);
#25968=AXIS2_PLACEMENT_3D('',#37123,#30229,#30230);
#25969=AXIS2_PLACEMENT_3D('',#37126,#30232,#30233);
#25970=AXIS2_PLACEMENT_3D('',#37131,#30235,#30236);
#25971=AXIS2_PLACEMENT_3D('',#37134,#30238,#30239);
#25972=AXIS2_PLACEMENT_3D('',#37139,#30241,#30242);
#25973=AXIS2_PLACEMENT_3D('',#37142,#30244,#30245);
#25974=AXIS2_PLACEMENT_3D('',#37144,#30246,#30247);
#25975=AXIS2_PLACEMENT_3D('',#37145,#30248,#30249);
#25976=AXIS2_PLACEMENT_3D('',#37146,#30250,#30251);
#25977=AXIS2_PLACEMENT_3D('',#37147,#30252,#30253);
#25978=AXIS2_PLACEMENT_3D('',#37149,#30254,#30255);
#25979=AXIS2_PLACEMENT_3D('',#37151,#30257,#30258);
#25980=AXIS2_PLACEMENT_3D('',#37153,#30259,#30260);
#25981=AXIS2_PLACEMENT_3D('',#37155,#30262,#30263);
#25982=AXIS2_PLACEMENT_3D('',#37157,#30264,#30265);
#25983=AXIS2_PLACEMENT_3D('',#37159,#30267,#30268);
#25984=AXIS2_PLACEMENT_3D('',#37165,#30272,#30273);
#25985=AXIS2_PLACEMENT_3D('',#37168,#30275,#30276);
#25986=AXIS2_PLACEMENT_3D('',#37169,#30277,#30278);
#25987=AXIS2_PLACEMENT_3D('',#37173,#30281,#30282);
#25988=AXIS2_PLACEMENT_3D('',#37174,#30283,#30284);
#25989=AXIS2_PLACEMENT_3D('',#37175,#30285,#30286);
#25990=AXIS2_PLACEMENT_3D('',#37181,#30290,#30291);
#25991=AXIS2_PLACEMENT_3D('',#37184,#30293,#30294);
#25992=AXIS2_PLACEMENT_3D('',#37185,#30295,#30296);
#25993=AXIS2_PLACEMENT_3D('',#37189,#30299,#30300);
#25994=AXIS2_PLACEMENT_3D('',#37190,#30301,#30302);
#25995=AXIS2_PLACEMENT_3D('',#37191,#30303,#30304);
#25996=AXIS2_PLACEMENT_3D('',#37197,#30308,#30309);
#25997=AXIS2_PLACEMENT_3D('',#37200,#30311,#30312);
#25998=AXIS2_PLACEMENT_3D('',#37201,#30313,#30314);
#25999=AXIS2_PLACEMENT_3D('',#37205,#30317,#30318);
#26000=AXIS2_PLACEMENT_3D('',#37206,#30319,#30320);
#26001=AXIS2_PLACEMENT_3D('',#37207,#30321,#30322);
#26002=AXIS2_PLACEMENT_3D('',#37213,#30326,#30327);
#26003=AXIS2_PLACEMENT_3D('',#37216,#30329,#30330);
#26004=AXIS2_PLACEMENT_3D('',#37217,#30331,#30332);
#26005=AXIS2_PLACEMENT_3D('',#37221,#30335,#30336);
#26006=AXIS2_PLACEMENT_3D('',#37222,#30337,#30338);
#26007=AXIS2_PLACEMENT_3D('',#37223,#30339,#30340);
#26008=AXIS2_PLACEMENT_3D('',#37229,#30344,#30345);
#26009=AXIS2_PLACEMENT_3D('',#37232,#30347,#30348);
#26010=AXIS2_PLACEMENT_3D('',#37233,#30349,#30350);
#26011=AXIS2_PLACEMENT_3D('',#37237,#30353,#30354);
#26012=AXIS2_PLACEMENT_3D('',#37238,#30355,#30356);
#26013=AXIS2_PLACEMENT_3D('',#37239,#30357,#30358);
#26014=AXIS2_PLACEMENT_3D('',#37245,#30362,#30363);
#26015=AXIS2_PLACEMENT_3D('',#37248,#30365,#30366);
#26016=AXIS2_PLACEMENT_3D('',#37249,#30367,#30368);
#26017=AXIS2_PLACEMENT_3D('',#37253,#30371,#30372);
#26018=AXIS2_PLACEMENT_3D('',#37254,#30373,#30374);
#26019=AXIS2_PLACEMENT_3D('',#37255,#30375,#30376);
#26020=AXIS2_PLACEMENT_3D('',#37257,#30377,#30378);
#26021=AXIS2_PLACEMENT_3D('',#37259,#30380,#30381);
#30182=DIRECTION('axis',(0.,0.,1.));
#30183=DIRECTION('refdir',(1.,0.,0.));
#30184=DIRECTION('center_axis',(0.,1.,0.));
#30185=DIRECTION('ref_axis',(-1.,0.,0.));
#30186=DIRECTION('',(0.,0.,-1.));
#30187=DIRECTION('',(1.,0.,0.));
#30188=DIRECTION('',(0.,0.,1.));
#30189=DIRECTION('',(-1.,0.,0.));
#30190=DIRECTION('center_axis',(0.,-1.,0.));
#30191=DIRECTION('ref_axis',(1.,0.,0.));
#30192=DIRECTION('',(0.,0.,1.));
#30193=DIRECTION('',(1.,0.,0.));
#30194=DIRECTION('',(0.,0.,1.));
#30195=DIRECTION('',(-1.,0.,0.));
#30196=DIRECTION('center_axis',(-1.,0.,0.));
#30197=DIRECTION('ref_axis',(0.,-1.,0.));
#30198=DIRECTION('',(0.,-1.,0.));
#30199=DIRECTION('',(0.,1.,0.));
#30200=DIRECTION('center_axis',(0.,0.,-1.));
#30201=DIRECTION('ref_axis',(-1.,0.,0.));
#30202=DIRECTION('center_axis',(0.,0.,1.));
#30203=DIRECTION('ref_axis',(1.,0.,0.));
#30204=DIRECTION('center_axis',(0.,0.,1.));
#30205=DIRECTION('ref_axis',(-1.,0.,0.));
#30206=DIRECTION('center_axis',(0.,0.,1.));
#30207=DIRECTION('ref_axis',(-1.,0.,0.));
#30208=DIRECTION('center_axis',(0.,0.,1.));
#30209=DIRECTION('ref_axis',(1.,0.,0.));
#30210=DIRECTION('',(1.,0.,0.));
#30211=DIRECTION('center_axis',(0.,0.,1.));
#30212=DIRECTION('ref_axis',(1.,2.06553120860494E-16,0.));
#30213=DIRECTION('',(-0.866025403784439,-0.5,0.));
#30214=DIRECTION('center_axis',(0.,0.,-1.));
#30215=DIRECTION('ref_axis',(1.,8.07434927000111E-16,0.));
#30216=DIRECTION('',(0.5,0.866025403784439,0.));
#30217=DIRECTION('center_axis',(0.,0.,1.));
#30218=DIRECTION('ref_axis',(0.5,0.866025403784439,0.));
#30219=DIRECTION('',(-2.77555756156289E-16,-1.,0.));
#30220=DIRECTION('center_axis',(0.,0.,-1.));
#30221=DIRECTION('ref_axis',(0.499999999999999,0.866025403784439,0.));
#30222=DIRECTION('',(-0.5,0.866025403784439,0.));
#30223=DIRECTION('center_axis',(0.,0.,1.));
#30224=DIRECTION('ref_axis',(-0.5,0.866025403784439,0.));
#30225=DIRECTION('',(0.866025403784438,-0.5,0.));
#30226=DIRECTION('center_axis',(0.,0.,-1.));
#30227=DIRECTION('ref_axis',(-0.500000000000001,0.866025403784438,0.));
#30228=DIRECTION('',(-1.,1.66533453693773E-16,0.));
#30229=DIRECTION('center_axis',(0.,0.,1.));
#30230=DIRECTION('ref_axis',(-1.,-5.16382802151235E-17,0.));
#30231=DIRECTION('',(0.866025403784439,0.5,0.));
#30232=DIRECTION('center_axis',(0.,0.,-1.));
#30233=DIRECTION('ref_axis',(-1.,-6.5604087818759E-16,0.));
#30234=DIRECTION('',(-0.5,-0.866025403784438,0.));
#30235=DIRECTION('center_axis',(0.,0.,1.));
#30236=DIRECTION('ref_axis',(-0.5,-0.866025403784438,0.));
#30237=DIRECTION('',(6.66133814775094E-16,1.,0.));
#30238=DIRECTION('center_axis',(0.,0.,-1.));
#30239=DIRECTION('ref_axis',(-0.5,-0.866025403784439,0.));
#30240=DIRECTION('',(0.499999999999999,-0.866025403784439,0.));
#30241=DIRECTION('center_axis',(0.,0.,1.));
#30242=DIRECTION('ref_axis',(0.5,-0.866025403784439,0.));
#30243=DIRECTION('',(-0.866025403784438,0.500000000000001,0.));
#30244=DIRECTION('center_axis',(0.,0.,-1.));
#30245=DIRECTION('ref_axis',(0.5,-0.866025403784439,0.));
#30246=DIRECTION('center_axis',(0.,0.,1.));
#30247=DIRECTION('ref_axis',(-1.,0.,0.));
#30248=DIRECTION('center_axis',(0.,0.,1.));
#30249=DIRECTION('ref_axis',(-1.,1.22464679914735E-16,0.));
#30250=DIRECTION('center_axis',(0.,0.,1.));
#30251=DIRECTION('ref_axis',(1.,0.,0.));
#30252=DIRECTION('center_axis',(0.,0.,-1.));
#30253=DIRECTION('ref_axis',(-1.,0.,0.));
#30254=DIRECTION('center_axis',(0.,0.,-1.));
#30255=DIRECTION('ref_axis',(-1.,0.,0.));
#30256=DIRECTION('',(0.,0.,-1.));
#30257=DIRECTION('center_axis',(0.,0.,-1.));
#30258=DIRECTION('ref_axis',(-1.,0.,0.));
#30259=DIRECTION('center_axis',(0.,0.,-1.));
#30260=DIRECTION('ref_axis',(-1.,0.,0.));
#30261=DIRECTION('',(0.,0.,-1.));
#30262=DIRECTION('center_axis',(0.,0.,-1.));
#30263=DIRECTION('ref_axis',(-1.,0.,0.));
#30264=DIRECTION('center_axis',(0.,0.,-1.));
#30265=DIRECTION('ref_axis',(-1.,0.,0.));
#30266=DIRECTION('',(0.,0.,-1.));
#30267=DIRECTION('center_axis',(-0.866025403784439,-0.499999999999999,0.));
#30268=DIRECTION('ref_axis',(0.499999999999999,-0.866025403784439,0.));
#30269=DIRECTION('',(0.,0.,1.));
#30270=DIRECTION('',(-0.499999999999999,0.866025403784439,0.));
#30271=DIRECTION('',(0.,0.,1.));
#30272=DIRECTION('center_axis',(0.,0.,1.));
#30273=DIRECTION('ref_axis',(0.5,-0.866025403784439,0.));
#30274=DIRECTION('',(0.,0.,1.));
#30275=DIRECTION('center_axis',(0.,0.,1.));
#30276=DIRECTION('ref_axis',(0.5,-0.866025403784439,0.));
#30277=DIRECTION('center_axis',(0.500000000000001,0.866025403784438,0.));
#30278=DIRECTION('ref_axis',(-0.866025403784438,0.500000000000001,0.));
#30279=DIRECTION('',(0.,0.,1.));
#30280=DIRECTION('',(0.866025403784438,-0.500000000000001,0.));
#30281=DIRECTION('center_axis',(0.,0.,1.));
#30282=DIRECTION('ref_axis',(0.5,-0.866025403784439,0.));
#30283=DIRECTION('center_axis',(0.,0.,-1.));
#30284=DIRECTION('ref_axis',(0.5,-0.866025403784439,0.));
#30285=DIRECTION('center_axis',(-0.866025403784438,0.5,0.));
#30286=DIRECTION('ref_axis',(-0.5,-0.866025403784438,0.));
#30287=DIRECTION('',(0.,0.,1.));
#30288=DIRECTION('',(0.5,0.866025403784438,0.));
#30289=DIRECTION('',(0.,0.,1.));
#30290=DIRECTION('center_axis',(0.,0.,1.));
#30291=DIRECTION('ref_axis',(-0.5,-0.866025403784439,0.));
#30292=DIRECTION('',(0.,0.,1.));
#30293=DIRECTION('center_axis',(0.,0.,1.));
#30294=DIRECTION('ref_axis',(-0.5,-0.866025403784439,0.));
#30295=DIRECTION('center_axis',(1.,-6.66133814775094E-16,0.));
#30296=DIRECTION('ref_axis',(6.66133814775094E-16,1.,0.));
#30297=DIRECTION('',(0.,0.,1.));
#30298=DIRECTION('',(-6.66133814775094E-16,-1.,0.));
#30299=DIRECTION('center_axis',(0.,0.,1.));
#30300=DIRECTION('ref_axis',(-0.5,-0.866025403784438,0.));
#30301=DIRECTION('center_axis',(0.,0.,-1.));
#30302=DIRECTION('ref_axis',(-0.5,-0.866025403784438,0.));
#30303=DIRECTION('center_axis',(1.66533453693773E-16,1.,0.));
#30304=DIRECTION('ref_axis',(-1.,1.66533453693773E-16,0.));
#30305=DIRECTION('',(0.,0.,1.));
#30306=DIRECTION('',(1.,-1.66533453693773E-16,0.));
#30307=DIRECTION('',(0.,0.,1.));
#30308=DIRECTION('center_axis',(0.,0.,1.));
#30309=DIRECTION('ref_axis',(-1.,-6.5604087818759E-16,0.));
#30310=DIRECTION('',(0.,0.,1.));
#30311=DIRECTION('center_axis',(0.,0.,1.));
#30312=DIRECTION('ref_axis',(-1.,-6.5604087818759E-16,0.));
#30313=DIRECTION('center_axis',(0.5,-0.866025403784439,0.));
#30314=DIRECTION('ref_axis',(0.866025403784439,0.5,0.));
#30315=DIRECTION('',(0.,0.,1.));
#30316=DIRECTION('',(-0.866025403784439,-0.5,0.));
#30317=DIRECTION('center_axis',(0.,0.,1.));
#30318=DIRECTION('ref_axis',(-1.,-5.16382802151235E-17,0.));
#30319=DIRECTION('center_axis',(0.,0.,-1.));
#30320=DIRECTION('ref_axis',(-1.,-5.16382802151235E-17,0.));
#30321=DIRECTION('center_axis',(0.866025403784439,0.5,0.));
#30322=DIRECTION('ref_axis',(-0.5,0.866025403784439,0.));
#30323=DIRECTION('',(0.,0.,1.));
#30324=DIRECTION('',(0.5,-0.866025403784439,0.));
#30325=DIRECTION('',(0.,0.,1.));
#30326=DIRECTION('center_axis',(0.,0.,1.));
#30327=DIRECTION('ref_axis',(-0.500000000000001,0.866025403784438,0.));
#30328=DIRECTION('',(0.,0.,1.));
#30329=DIRECTION('center_axis',(0.,0.,1.));
#30330=DIRECTION('ref_axis',(-0.500000000000001,0.866025403784438,0.));
#30331=DIRECTION('center_axis',(-0.5,-0.866025403784438,0.));
#30332=DIRECTION('ref_axis',(0.866025403784438,-0.5,0.));
#30333=DIRECTION('',(0.,0.,1.));
#30334=DIRECTION('',(-0.866025403784438,0.5,0.));
#30335=DIRECTION('center_axis',(0.,0.,1.));
#30336=DIRECTION('ref_axis',(-0.5,0.866025403784439,0.));
#30337=DIRECTION('center_axis',(0.,0.,-1.));
#30338=DIRECTION('ref_axis',(-0.5,0.866025403784439,0.));
#30339=DIRECTION('center_axis',(0.866025403784439,-0.5,0.));
#30340=DIRECTION('ref_axis',(0.5,0.866025403784439,0.));
#30341=DIRECTION('',(0.,0.,1.));
#30342=DIRECTION('',(-0.5,-0.866025403784439,0.));
#30343=DIRECTION('',(0.,0.,1.));
#30344=DIRECTION('center_axis',(0.,0.,1.));
#30345=DIRECTION('ref_axis',(0.499999999999999,0.866025403784439,0.));
#30346=DIRECTION('',(0.,0.,1.));
#30347=DIRECTION('center_axis',(0.,0.,1.));
#30348=DIRECTION('ref_axis',(0.499999999999999,0.866025403784439,0.));
#30349=DIRECTION('center_axis',(-1.,2.77555756156289E-16,0.));
#30350=DIRECTION('ref_axis',(-2.77555756156289E-16,-1.,0.));
#30351=DIRECTION('',(0.,0.,1.));
#30352=DIRECTION('',(2.77555756156289E-16,1.,0.));
#30353=DIRECTION('center_axis',(0.,0.,1.));
#30354=DIRECTION('ref_axis',(0.5,0.866025403784439,0.));
#30355=DIRECTION('center_axis',(0.,0.,-1.));
#30356=DIRECTION('ref_axis',(0.5,0.866025403784439,0.));
#30357=DIRECTION('center_axis',(0.,-1.,0.));
#30358=DIRECTION('ref_axis',(1.,0.,0.));
#30359=DIRECTION('',(0.,0.,1.));
#30360=DIRECTION('',(-1.,0.,0.));
#30361=DIRECTION('',(0.,0.,1.));
#30362=DIRECTION('center_axis',(0.,0.,1.));
#30363=DIRECTION('ref_axis',(1.,8.07434927000111E-16,0.));
#30364=DIRECTION('',(0.,0.,1.));
#30365=DIRECTION('center_axis',(0.,0.,1.));
#30366=DIRECTION('ref_axis',(1.,8.07434927000111E-16,0.));
#30367=DIRECTION('center_axis',(-0.5,0.866025403784439,0.));
#30368=DIRECTION('ref_axis',(-0.866025403784439,-0.5,0.));
#30369=DIRECTION('',(0.,0.,1.));
#30370=DIRECTION('',(0.866025403784439,0.5,0.));
#30371=DIRECTION('center_axis',(0.,0.,1.));
#30372=DIRECTION('ref_axis',(1.,2.06553120860494E-16,0.));
#30373=DIRECTION('center_axis',(0.,0.,-1.));
#30374=DIRECTION('ref_axis',(1.,2.06553120860494E-16,0.));
#30375=DIRECTION('center_axis',(0.,0.,1.));
#30376=DIRECTION('ref_axis',(1.,0.,0.));
#30377=DIRECTION('center_axis',(0.,0.,1.));
#30378=DIRECTION('ref_axis',(1.,0.,0.));
#30379=DIRECTION('',(0.,0.,-1.));
#30380=DIRECTION('center_axis',(0.,0.,1.));
#30381=DIRECTION('ref_axis',(1.,0.,0.));
#37065=CARTESIAN_POINT('',(0.,0.,0.));
#37066=CARTESIAN_POINT('Origin',(2.4,0.06,10.91));
#37067=CARTESIAN_POINT('',(2.34923391768466,0.06,10.96));
#37068=CARTESIAN_POINT('',(2.34923391768466,0.06,10.91));
#37069=CARTESIAN_POINT('',(2.34923391768466,0.06,10.935));
#37070=CARTESIAN_POINT('',(2.23,0.06,10.96));
#37071=CARTESIAN_POINT('',(1.30125,0.06,10.96));
#37072=CARTESIAN_POINT('',(2.23,0.06,10.91));
#37073=CARTESIAN_POINT('',(2.23,0.06,10.91));
#37074=CARTESIAN_POINT('',(2.375,0.06,10.91));
#37075=CARTESIAN_POINT('Origin',(2.23,-0.06,10.91));
#37076=CARTESIAN_POINT('',(2.34923391768466,-0.06,10.91));
#37077=CARTESIAN_POINT('',(2.34923391768466,-0.06,10.96));
#37078=CARTESIAN_POINT('',(2.34923391768466,-0.06,10.935));
#37079=CARTESIAN_POINT('',(2.23,-0.06,10.91));
#37080=CARTESIAN_POINT('',(2.29,-0.06,10.91));
#37081=CARTESIAN_POINT('',(2.23,-0.06,10.96));
#37082=CARTESIAN_POINT('',(2.23,-0.06,10.91));
#37083=CARTESIAN_POINT('',(1.21625,-0.06,10.96));
#37084=CARTESIAN_POINT('Origin',(2.23,0.06,10.91));
#37085=CARTESIAN_POINT('',(2.23,0.03,10.91));
#37086=CARTESIAN_POINT('',(2.23,0.03,10.96));
#37087=CARTESIAN_POINT('Origin',(2.35,0.,10.91));
#37088=CARTESIAN_POINT('Origin',(0.,0.,10.91));
#37089=CARTESIAN_POINT('',(-0.185,-0.476313972081441,10.91));
#37090=CARTESIAN_POINT('Origin',(-0.275,-0.476313972081441,10.91));
#37091=CARTESIAN_POINT('',(0.64,1.10218211923262E-17,10.91));
#37092=CARTESIAN_POINT('Origin',(0.55,0.,10.91));
#37093=CARTESIAN_POINT('',(-0.2025,-2.47990976827339E-17,10.91));
#37094=CARTESIAN_POINT('Origin',(0.,0.,10.91));
#37095=CARTESIAN_POINT('',(1.1,0.,10.91));
#37096=CARTESIAN_POINT('',(2.15,0.,10.91));
#37097=CARTESIAN_POINT('',(1.725,0.,10.91));
#37098=CARTESIAN_POINT('',(1.86195461813654,1.075,10.91));
#37099=CARTESIAN_POINT('Origin',(-2.22044604925031E-15,-4.44089209850063E-16,
10.91));
#37100=CARTESIAN_POINT('',(0.952627944162883,0.55,10.91));
#37101=CARTESIAN_POINT('',(1.81222730906827,1.04628992472336,10.91));
#37102=CARTESIAN_POINT('Origin',(-3.33066907387547E-15,-8.88178419700125E-16,
10.91));
#37103=CARTESIAN_POINT('',(0.55,0.952627944162883,10.91));
#37104=CARTESIAN_POINT('',(1.075,1.86195461813654,10.91));
#37105=CARTESIAN_POINT('',(0.56875,0.985103896804799,10.91));
#37106=CARTESIAN_POINT('',(5.55111512312578E-16,2.15,10.91));
#37107=CARTESIAN_POINT('Origin',(-7.25630487348444E-16,-2.1450072913086E-15,
10.91));
#37108=CARTESIAN_POINT('',(2.77555756156289E-16,1.1,10.91));
#37109=CARTESIAN_POINT('',(2.22044604925031E-16,1.075,10.91));
#37110=CARTESIAN_POINT('Origin',(-8.9614946238431E-16,-3.32853323942541E-15,
10.91));
#37111=CARTESIAN_POINT('',(-0.55,0.952627944162883,10.91));
#37112=CARTESIAN_POINT('',(-1.075,1.86195461813654,10.91));
#37113=CARTESIAN_POINT('',(0.0187499999999997,-0.0324759526419162,10.91));
#37114=CARTESIAN_POINT('',(-1.86195461813654,1.075,10.91));
#37115=CARTESIAN_POINT('Origin',(1.49481556190187E-15,-1.70091808145853E-15,
10.91));
#37116=CARTESIAN_POINT('',(-0.952627944162882,0.55,10.91));
#37117=CARTESIAN_POINT('',(-0.0497273090682718,0.0287100752766422,10.91));
#37118=CARTESIAN_POINT('Origin',(2.43451961149116E-15,-2.44035481972528E-15,
10.91));
#37119=CARTESIAN_POINT('',(-1.1,1.66533453693773E-16,10.91));
#37120=CARTESIAN_POINT('',(-2.15,3.33066907387547E-16,10.91));
#37121=CARTESIAN_POINT('',(0.625,-1.20736753927986E-16,10.91));
#37122=CARTESIAN_POINT('',(-1.86195461813654,-1.075,10.91));
#37123=CARTESIAN_POINT('Origin',(2.22044604925031E-15,4.44089209850062E-16,
10.91));
#37124=CARTESIAN_POINT('',(-0.952627944162883,-0.55,10.91));
#37125=CARTESIAN_POINT('',(-0.0497273090682713,-0.0287100752766424,10.91));
#37126=CARTESIAN_POINT('Origin',(3.33066907387547E-15,8.88178419700125E-16,
10.91));
#37127=CARTESIAN_POINT('',(-0.55,-0.952627944162882,10.91));
#37128=CARTESIAN_POINT('',(-1.075,-1.86195461813654,10.91));
#37129=CARTESIAN_POINT('',(0.0187500000000005,0.0324759526419168,10.91));
#37130=CARTESIAN_POINT('',(-1.33226762955019E-15,-2.15,10.91));
#37131=CARTESIAN_POINT('Origin',(7.25630487348445E-16,2.14500729130859E-15,
10.91));
#37132=CARTESIAN_POINT('',(-6.66133814775094E-16,-1.1,10.91));
#37133=CARTESIAN_POINT('',(-6.66133814775094E-16,-1.075,10.91));
#37134=CARTESIAN_POINT('Origin',(8.96149462384311E-16,3.32853323942541E-15,
10.91));
#37135=CARTESIAN_POINT('',(0.549999999999999,-0.952627944162883,10.91));
#37136=CARTESIAN_POINT('',(1.075,-1.86195461813654,10.91));
#37137=CARTESIAN_POINT('',(0.568749999999999,-0.985103896804799,10.91));
#37138=CARTESIAN_POINT('',(1.86195461813654,-1.075,10.91));
#37139=CARTESIAN_POINT('Origin',(-1.49481556190187E-15,1.70091808145853E-15,
10.91));
#37140=CARTESIAN_POINT('',(0.952627944162882,-0.550000000000001,10.91));
#37141=CARTESIAN_POINT('',(1.81222730906827,-1.04628992472336,10.91));
#37142=CARTESIAN_POINT('Origin',(-2.43451961149116E-15,2.44035481972529E-15,
10.91));
#37143=CARTESIAN_POINT('',(-0.185,0.476313972081441,10.91));
#37144=CARTESIAN_POINT('Origin',(-0.275,0.476313972081441,10.91));
#37145=CARTESIAN_POINT('Origin',(0.,0.,10.935));
#37146=CARTESIAN_POINT('Origin',(0.,0.,10.96));
#37147=CARTESIAN_POINT('Origin',(-0.275,-0.476313972081441,10.91));
#37148=CARTESIAN_POINT('',(-0.185,-0.476313972081441,10.96));
#37149=CARTESIAN_POINT('Origin',(-0.275,-0.476313972081441,10.96));
#37150=CARTESIAN_POINT('',(-0.185,-0.476313972081441,10.91));
#37151=CARTESIAN_POINT('Origin',(-0.275,0.476313972081441,10.91));
#37152=CARTESIAN_POINT('',(-0.185,0.476313972081441,10.96));
#37153=CARTESIAN_POINT('Origin',(-0.275,0.476313972081441,10.96));
#37154=CARTESIAN_POINT('',(-0.185,0.476313972081441,10.91));
#37155=CARTESIAN_POINT('Origin',(0.55,0.,10.91));
#37156=CARTESIAN_POINT('',(0.64,-1.10218211923262E-17,10.96));
#37157=CARTESIAN_POINT('Origin',(0.55,0.,10.96));
#37158=CARTESIAN_POINT('',(0.64,-1.10218211923262E-17,10.91));
#37159=CARTESIAN_POINT('Origin',(0.549999999999999,-0.952627944162883,10.91));
#37160=CARTESIAN_POINT('',(0.549999999999999,-0.952627944162883,10.96));
#37161=CARTESIAN_POINT('',(0.549999999999999,-0.952627944162883,10.91));
#37162=CARTESIAN_POINT('',(1.075,-1.86195461813654,10.96));
#37163=CARTESIAN_POINT('',(0.3003125,-0.520156508148029,10.96));
#37164=CARTESIAN_POINT('',(1.075,-1.86195461813654,10.91));
#37165=CARTESIAN_POINT('Origin',(-2.43451961149116E-15,2.44035481972529E-15,
10.91));
#37166=CARTESIAN_POINT('',(0.952627944162882,-0.550000000000001,10.96));
#37167=CARTESIAN_POINT('',(0.952627944162882,-0.550000000000001,10.91));
#37168=CARTESIAN_POINT('Origin',(-2.43451961149116E-15,2.44035481972529E-15,
10.96));
#37169=CARTESIAN_POINT('Origin',(1.86195461813654,-1.075,10.91));
#37170=CARTESIAN_POINT('',(1.86195461813654,-1.075,10.96));
#37171=CARTESIAN_POINT('',(1.86195461813654,-1.075,10.91));
#37172=CARTESIAN_POINT('',(1.00691480906827,-0.581342536066588,10.96));
#37173=CARTESIAN_POINT('Origin',(-1.49481556190187E-15,1.70091808145853E-15,
10.91));
#37174=CARTESIAN_POINT('Origin',(-1.49481556190187E-15,1.70091808145853E-15,
10.96));
#37175=CARTESIAN_POINT('Origin',(-0.55,-0.952627944162882,10.91));
#37176=CARTESIAN_POINT('',(-0.55,-0.952627944162882,10.96));
#37177=CARTESIAN_POINT('',(-0.55,-0.952627944162882,10.91));
#37178=CARTESIAN_POINT('',(-1.075,-1.86195461813654,10.96));
#37179=CARTESIAN_POINT('',(-0.2496875,-0.432471436014854,10.96));
#37180=CARTESIAN_POINT('',(-1.075,-1.86195461813654,10.91));
#37181=CARTESIAN_POINT('Origin',(8.96149462384311E-16,3.32853323942541E-15,
10.91));
#37182=CARTESIAN_POINT('',(-6.66133814775094E-16,-1.1,10.96));
#37183=CARTESIAN_POINT('',(-6.66133814775094E-16,-1.1,10.91));
#37184=CARTESIAN_POINT('Origin',(8.96149462384311E-16,3.32853323942541E-15,
10.96));
#37185=CARTESIAN_POINT('Origin',(-1.33226762955019E-15,-2.15,10.91));
#37186=CARTESIAN_POINT('',(-1.33226762955019E-15,-2.15,10.96));
#37187=CARTESIAN_POINT('',(-1.33226762955019E-15,-2.15,10.91));
#37188=CARTESIAN_POINT('',(-6.10622663543836E-16,-1.075,10.96));
#37189=CARTESIAN_POINT('Origin',(7.25630487348445E-16,2.14500729130859E-15,
10.91));
#37190=CARTESIAN_POINT('Origin',(7.25630487348445E-16,2.14500729130859E-15,
10.96));
#37191=CARTESIAN_POINT('Origin',(-1.1,1.66533453693773E-16,10.91));
#37192=CARTESIAN_POINT('',(-1.1,1.66533453693773E-16,10.96));
#37193=CARTESIAN_POINT('',(-1.1,1.66533453693773E-16,10.91));
#37194=CARTESIAN_POINT('',(-2.15,3.33066907387547E-16,10.96));
#37195=CARTESIAN_POINT('',(-0.44875,5.80785419757035E-17,10.96));
#37196=CARTESIAN_POINT('',(-2.15,3.33066907387547E-16,10.91));
#37197=CARTESIAN_POINT('Origin',(3.33066907387547E-15,8.88178419700125E-16,
10.91));
#37198=CARTESIAN_POINT('',(-0.952627944162883,-0.55,10.96));
#37199=CARTESIAN_POINT('',(-0.952627944162883,-0.55,10.91));
#37200=CARTESIAN_POINT('Origin',(3.33066907387547E-15,8.88178419700125E-16,
10.96));
#37201=CARTESIAN_POINT('Origin',(-1.86195461813654,-1.075,10.91));
#37202=CARTESIAN_POINT('',(-1.86195461813654,-1.075,10.96));
#37203=CARTESIAN_POINT('',(-1.86195461813654,-1.075,10.91));
#37204=CARTESIAN_POINT('',(-0.855039809068272,-0.493657463933413,10.96));
#37205=CARTESIAN_POINT('Origin',(2.22044604925031E-15,4.44089209850062E-16,
10.91));
#37206=CARTESIAN_POINT('Origin',(2.22044604925031E-15,4.44089209850062E-16,
10.96));
#37207=CARTESIAN_POINT('Origin',(-0.55,0.952627944162883,10.91));
#37208=CARTESIAN_POINT('',(-0.55,0.952627944162883,10.96));
#37209=CARTESIAN_POINT('',(-0.55,0.952627944162883,10.91));
#37210=CARTESIAN_POINT('',(-1.075,1.86195461813654,10.96));
#37211=CARTESIAN_POINT('',(-0.2496875,0.432471436014854,10.96));
#37212=CARTESIAN_POINT('',(-1.075,1.86195461813654,10.91));
#37213=CARTESIAN_POINT('Origin',(2.43451961149116E-15,-2.44035481972528E-15,
10.91));
#37214=CARTESIAN_POINT('',(-0.952627944162882,0.55,10.96));
#37215=CARTESIAN_POINT('',(-0.952627944162882,0.55,10.91));
#37216=CARTESIAN_POINT('Origin',(2.43451961149116E-15,-2.44035481972528E-15,
10.96));
#37217=CARTESIAN_POINT('Origin',(-1.86195461813654,1.075,10.91));
#37218=CARTESIAN_POINT('',(-1.86195461813654,1.075,10.96));
#37219=CARTESIAN_POINT('',(-1.86195461813654,1.075,10.91));
#37220=CARTESIAN_POINT('',(-0.855039809068271,0.493657463933413,10.96));
#37221=CARTESIAN_POINT('Origin',(1.49481556190187E-15,-1.70091808145853E-15,
10.91));
#37222=CARTESIAN_POINT('Origin',(1.49481556190187E-15,-1.70091808145853E-15,
10.96));
#37223=CARTESIAN_POINT('Origin',(0.55,0.952627944162883,10.91));
#37224=CARTESIAN_POINT('',(0.55,0.952627944162883,10.96));
#37225=CARTESIAN_POINT('',(0.55,0.952627944162883,10.91));
#37226=CARTESIAN_POINT('',(1.075,1.86195461813654,10.96));
#37227=CARTESIAN_POINT('',(0.3003125,0.520156508148028,10.96));
#37228=CARTESIAN_POINT('',(1.075,1.86195461813654,10.91));
#37229=CARTESIAN_POINT('Origin',(-8.9614946238431E-16,-3.32853323942541E-15,
10.91));
#37230=CARTESIAN_POINT('',(2.77555756156289E-16,1.1,10.96));
#37231=CARTESIAN_POINT('',(2.77555756156289E-16,1.1,10.91));
#37232=CARTESIAN_POINT('Origin',(-8.9614946238431E-16,-3.32853323942541E-15,
10.96));
#37233=CARTESIAN_POINT('Origin',(5.55111512312578E-16,2.15,10.91));
#37234=CARTESIAN_POINT('',(5.55111512312578E-16,2.15,10.96));
#37235=CARTESIAN_POINT('',(5.55111512312578E-16,2.15,10.91));
#37236=CARTESIAN_POINT('',(2.4980018054066E-16,1.075,10.96));
#37237=CARTESIAN_POINT('Origin',(-7.25630487348444E-16,-2.1450072913086E-15,
10.91));
#37238=CARTESIAN_POINT('Origin',(-7.25630487348444E-16,-2.1450072913086E-15,
10.96));
#37239=CARTESIAN_POINT('Origin',(1.1,0.,10.91));
#37240=CARTESIAN_POINT('',(1.1,0.,10.96));
#37241=CARTESIAN_POINT('',(1.1,0.,10.91));
#37242=CARTESIAN_POINT('',(2.15,0.,10.96));
#37243=CARTESIAN_POINT('',(0.65125,0.,10.96));
#37244=CARTESIAN_POINT('',(2.15,0.,10.91));
#37245=CARTESIAN_POINT('Origin',(-3.33066907387547E-15,-8.88178419700125E-16,
10.91));
#37246=CARTESIAN_POINT('',(0.952627944162883,0.55,10.96));
#37247=CARTESIAN_POINT('',(0.952627944162883,0.55,10.91));
#37248=CARTESIAN_POINT('Origin',(-3.33066907387547E-15,-8.88178419700125E-16,
10.96));
#37249=CARTESIAN_POINT('Origin',(1.86195461813654,1.075,10.91));
#37250=CARTESIAN_POINT('',(1.86195461813654,1.075,10.96));
#37251=CARTESIAN_POINT('',(1.86195461813654,1.075,10.91));
#37252=CARTESIAN_POINT('',(1.00691480906827,0.581342536066587,10.96));
#37253=CARTESIAN_POINT('Origin',(-2.22044604925031E-15,-4.44089209850063E-16,
10.91));
#37254=CARTESIAN_POINT('Origin',(-2.22044604925031E-15,-4.44089209850063E-16,
10.96));
#37255=CARTESIAN_POINT('Origin',(0.,0.,10.935));
#37256=CARTESIAN_POINT('',(-0.2025,-2.47990976827339E-17,10.96));
#37257=CARTESIAN_POINT('Origin',(0.,0.,10.96));
#37258=CARTESIAN_POINT('',(-0.2025,-2.47990976827339E-17,10.935));
#37259=CARTESIAN_POINT('Origin',(0.2025,0.,10.96));
#54969=UNCERTAINTY_MEASURE_WITH_UNIT(LENGTH_MEASURE(0.001),#55003,
'DISTANCE_ACCURACY_VALUE',
'Maximum model space distance between geometric entities at asserted c
onnectivities');
#54980=UNCERTAINTY_MEASURE_WITH_UNIT(LENGTH_MEASURE(0.001),#55003,
'DISTANCE_ACCURACY_VALUE',
'Maximum model space distance between geometric entities at asserted c
onnectivities');
#54991=(
GEOMETRIC_REPRESENTATION_CONTEXT(3)
GLOBAL_UNCERTAINTY_ASSIGNED_CONTEXT((#54969))
GLOBAL_UNIT_ASSIGNED_CONTEXT((#55003,#55005,#55006))
REPRESENTATION_CONTEXT('','3D')
);
#55002=(
GEOMETRIC_REPRESENTATION_CONTEXT(3)
GLOBAL_UNCERTAINTY_ASSIGNED_CONTEXT((#54980))
GLOBAL_UNIT_ASSIGNED_CONTEXT((#55003,#55005,#55006))
REPRESENTATION_CONTEXT('','3D')
);
#55003=(
LENGTH_UNIT()
NAMED_UNIT(*)
SI_UNIT(.CENTI.,.METRE.)
);
#55005=(
NAMED_UNIT(*)
PLANE_ANGLE_UNIT()
SI_UNIT($,.RADIAN.)
);
#55006=(
NAMED_UNIT(*)
SI_UNIT($,.STERADIAN.)
SOLID_ANGLE_UNIT()
);
#55017=SHAPE_DEFINITION_REPRESENTATION(#55038,#55113);
#55038=PRODUCT_DEFINITION_SHAPE('',$,#55135);
#55113=SHAPE_REPRESENTATION('',(#25953),#54991);
#55124=PRODUCT_DEFINITION_CONTEXT('part definition',#55189,'design');
#55135=PRODUCT_DEFINITION('2026-10-18-23-36-26-322',
'10_Photo-Etched_Slotted_Chopper_Disc_D47x0.5',#55156,#55124);
#55156=PRODUCT_DEFINITION_FORMATION('',$,#55201);
#55189=APPLICATION_CONTEXT(
'Core Data for Automotive Mechanical Design Process');
#55190=PRODUCT_CONTEXT('part definition',#55189,'mechanical');
#55201=PRODUCT('2026-10-18-23-36-26-322',
'10_Photo-Etched_Slotted_Chopper_Disc_D47x0.5',$,(#55190));
#55373=COLOUR_RGB('Sky Blue',0.24,0.69,0.87);
#55374=FILL_AREA_STYLE_COLOUR('',#55373);
#55375=FILL_AREA_STYLE('',(#55374));
#55376=SURFACE_STYLE_FILL_AREA(#55375);
#55377=SURFACE_SIDE_STYLE('',(#55376));
#55378=SURFACE_STYLE_USAGE(.BOTH.,#55377);
#55379=PRESENTATION_STYLE_ASSIGNMENT((#55378));
ENDSEC;
END-ISO-10303-21;
